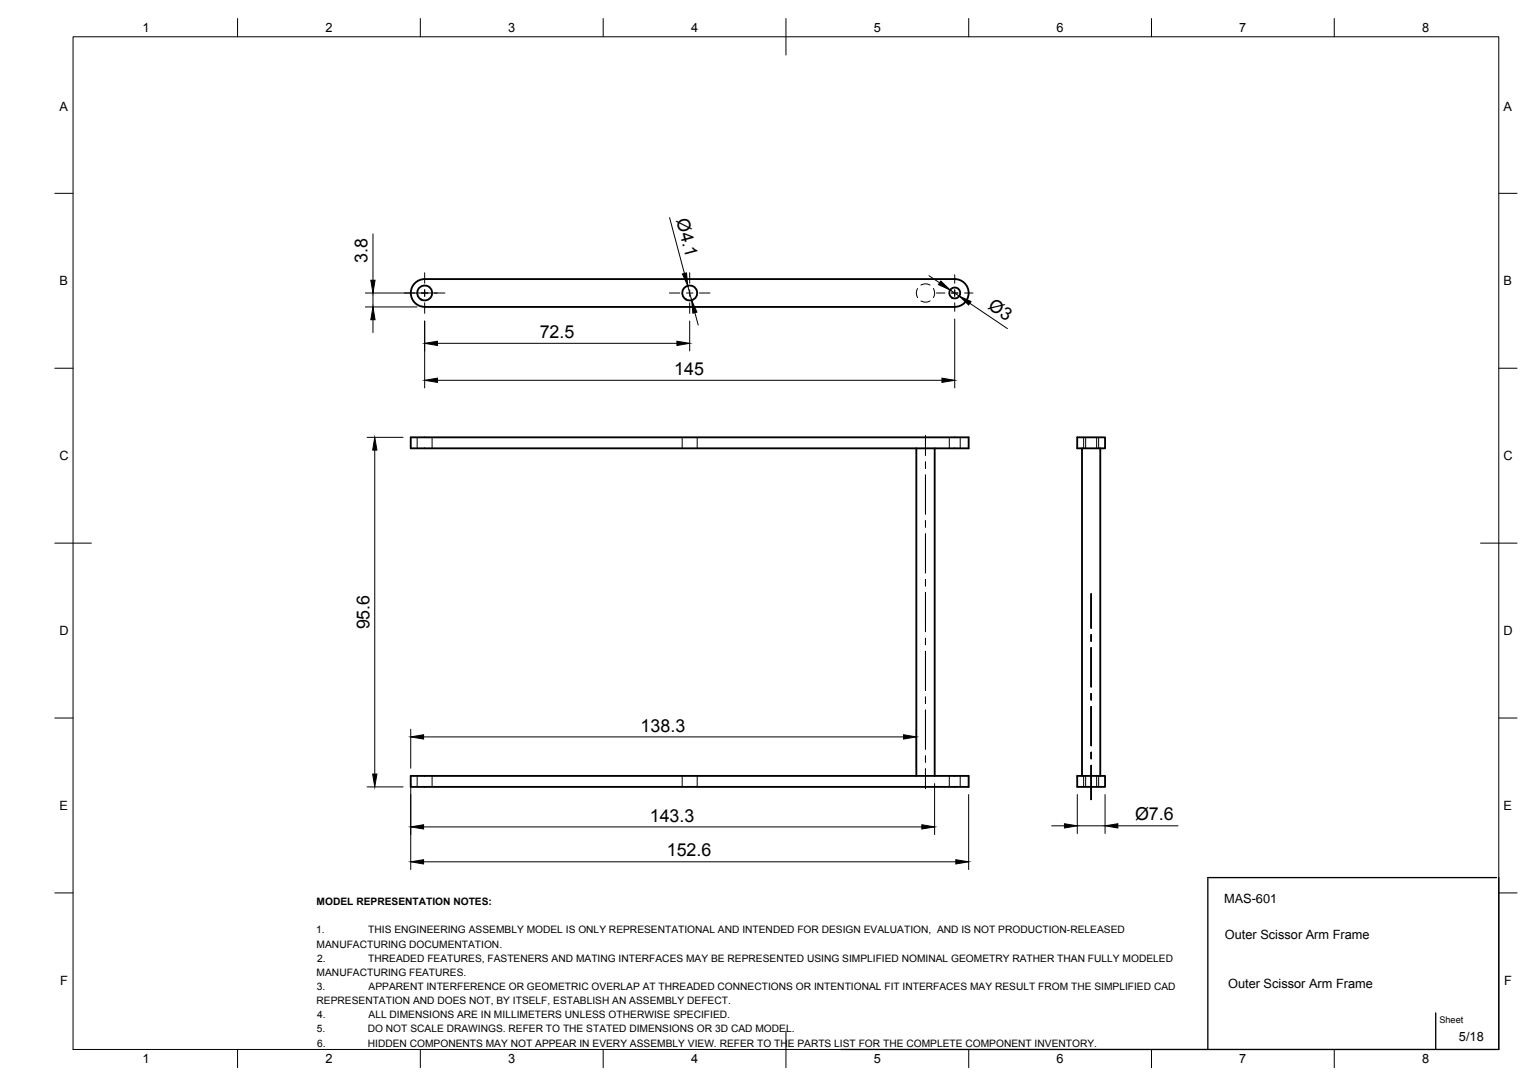
ISO-10303-21;
HEADER;
FILE_DESCRIPTION((''),'2;1');
FILE_NAME('Outer Scissor Arm Frame.step','2026-10-06T07:37:42+05:00',(''),(''),'','','');
FILE_SCHEMA (('AUTOMOTIVE_DESIGN { 1 0 10303 214 3 1 1 }'));
ENDSEC;
DATA;
#10=MECHANICAL_DESIGN_GEOMETRIC_PRESENTATION_REPRESENTATION('',(#375),#18757);
#341=SHAPE_REPRESENTATION_RELATIONSHIP('SRR','None',#18859,#358) ;
#358=ADVANCED_BREP_SHAPE_REPRESENTATION('',(#392),#18742) ;
#375=STYLED_ITEM('',(#18953),#392) ;
#392=MANIFOLD_SOLID_BREP('Outer Scissor Arm Frame',#9544) ;
#538=CYLINDRICAL_SURFACE('',#9984,2.5) ;
#539=CYLINDRICAL_SURFACE('',#9987,1.5) ;
#540=CYLINDRICAL_SURFACE('',#9990,2.05) ;
#541=CYLINDRICAL_SURFACE('',#9993,2.05) ;
#542=CYLINDRICAL_SURFACE('',#9997,3.8) ;
#543=CYLINDRICAL_SURFACE('',#10001,3.8) ;
#544=CYLINDRICAL_SURFACE('',#10006,1.5) ;
#545=CYLINDRICAL_SURFACE('',#10009,2.05) ;
#546=CYLINDRICAL_SURFACE('',#10012,2.05) ;
#547=CYLINDRICAL_SURFACE('',#10016,3.8) ;
#548=CYLINDRICAL_SURFACE('',#10020,3.8) ;
#682=FACE_BOUND('',#1785,.T.) ;
#683=FACE_BOUND('',#1786,.T.) ;
#684=FACE_BOUND('',#1787,.T.) ;
#685=FACE_BOUND('',#1788,.T.) ;
#686=FACE_BOUND('',#1790,.T.) ;
#687=FACE_BOUND('',#1791,.T.) ;
#688=FACE_BOUND('',#1792,.T.) ;
#689=FACE_BOUND('',#1801,.T.) ;
#690=FACE_BOUND('',#1802,.T.) ;
#691=FACE_BOUND('',#1803,.T.) ;
#692=FACE_BOUND('',#1805,.T.) ;
#693=FACE_BOUND('',#1806,.T.) ;
#694=FACE_BOUND('',#1807,.T.) ;
#695=FACE_BOUND('',#1808,.T.) ;
#840=PLANE('',#9996) ;
#841=PLANE('',#10000) ;
#842=PLANE('',#10004) ;
#843=PLANE('',#10005) ;
#844=PLANE('',#10015) ;
#845=PLANE('',#10019) ;
#846=PLANE('',#10023) ;
#847=PLANE('',#10024) ;
#1226=FACE_OUTER_BOUND('',#1776,.T.) ;
#1227=FACE_OUTER_BOUND('',#1777,.T.) ;
#1228=FACE_OUTER_BOUND('',#1778,.T.) ;
#1229=FACE_OUTER_BOUND('',#1779,.T.) ;
#1230=FACE_OUTER_BOUND('',#1780,.T.) ;
#1231=FACE_OUTER_BOUND('',#1781,.T.) ;
#1232=FACE_OUTER_BOUND('',#1782,.T.) ;
#1233=FACE_OUTER_BOUND('',#1783,.T.) ;
#1234=FACE_OUTER_BOUND('',#1784,.T.) ;
#1235=FACE_OUTER_BOUND('',#1789,.T.) ;
#1236=FACE_OUTER_BOUND('',#1793,.T.) ;
#1237=FACE_OUTER_BOUND('',#1794,.T.) ;
#1238=FACE_OUTER_BOUND('',#1795,.T.) ;
#1239=FACE_OUTER_BOUND('',#1796,.T.) ;
#1240=FACE_OUTER_BOUND('',#1797,.T.) ;
#1241=FACE_OUTER_BOUND('',#1798,.T.) ;
#1242=FACE_OUTER_BOUND('',#1799,.T.) ;
#1243=FACE_OUTER_BOUND('',#1800,.T.) ;
#1244=FACE_OUTER_BOUND('',#1804,.T.) ;
#1776=EDGE_LOOP('',(#7071,#7072,#7073,#7074)) ;
#1777=EDGE_LOOP('',(#7075,#7076,#7077,#7078)) ;
#1778=EDGE_LOOP('',(#7079,#7080,#7081,#7082)) ;
#1779=EDGE_LOOP('',(#7083,#7084,#7085,#7086)) ;
#1780=EDGE_LOOP('',(#7087,#7088,#7089,#7090)) ;
#1781=EDGE_LOOP('',(#7091,#7092,#7093,#7094)) ;
#1782=EDGE_LOOP('',(#7095,#7096,#7097,#7098)) ;
#1783=EDGE_LOOP('',(#7099,#7100,#7101,#7102)) ;
#1784=EDGE_LOOP('',(#7103,#7104,#7105,#7106)) ;
#1785=EDGE_LOOP('',(#7107)) ;
#1786=EDGE_LOOP('',(#7108)) ;
#1787=EDGE_LOOP('',(#7109)) ;
#1788=EDGE_LOOP('',(#7110)) ;
#1789=EDGE_LOOP('',(#7111,#7112,#7113,#7114)) ;
#1790=EDGE_LOOP('',(#7115)) ;
#1791=EDGE_LOOP('',(#7116)) ;
#1792=EDGE_LOOP('',(#7117)) ;
#1793=EDGE_LOOP('',(#7118,#7119,#7120,#7121)) ;
#1794=EDGE_LOOP('',(#7122,#7123,#7124,#7125)) ;
#1795=EDGE_LOOP('',(#7126,#7127,#7128,#7129)) ;
#1796=EDGE_LOOP('',(#7130,#7131,#7132,#7133)) ;
#1797=EDGE_LOOP('',(#7134,#7135,#7136,#7137)) ;
#1798=EDGE_LOOP('',(#7138,#7139,#7140,#7141)) ;
#1799=EDGE_LOOP('',(#7142,#7143,#7144,#7145)) ;
#1800=EDGE_LOOP('',(#7146,#7147,#7148,#7149)) ;
#1801=EDGE_LOOP('',(#7150)) ;
#1802=EDGE_LOOP('',(#7151)) ;
#1803=EDGE_LOOP('',(#7152)) ;
#1804=EDGE_LOOP('',(#7153,#7154,#7155,#7156)) ;
#1805=EDGE_LOOP('',(#7157)) ;
#1806=EDGE_LOOP('',(#7158)) ;
#1807=EDGE_LOOP('',(#7159)) ;
#1808=EDGE_LOOP('',(#7160)) ;
#2491=LINE('',#14387,#3262) ;
#2492=LINE('',#14393,#3263) ;
#2493=LINE('',#14399,#3264) ;
#2494=LINE('',#14405,#3265) ;
#2495=LINE('',#14410,#3266) ;
#2496=LINE('',#14412,#3267) ;
#2497=LINE('',#14414,#3268) ;
#2498=LINE('',#14415,#3269) ;
#2499=LINE('',#14421,#3270) ;
#2500=LINE('',#14424,#3271) ;
#2501=LINE('',#14426,#3272) ;
#2502=LINE('',#14427,#3273) ;
#2503=LINE('',#14437,#3274) ;
#2504=LINE('',#14443,#3275) ;
#2505=LINE('',#14449,#3276) ;
#2506=LINE('',#14454,#3277) ;
#2507=LINE('',#14456,#3278) ;
#2508=LINE('',#14458,#3279) ;
#2509=LINE('',#14459,#3280) ;
#2510=LINE('',#14465,#3281) ;
#2511=LINE('',#14468,#3282) ;
#2512=LINE('',#14470,#3283) ;
#2513=LINE('',#14471,#3284) ;
#3262=VECTOR('',#11451,2.5) ;
#3263=VECTOR('',#11458,1.5) ;
#3264=VECTOR('',#11465,2.05) ;
#3265=VECTOR('',#11472,2.05) ;
#3266=VECTOR('',#11477,10.) ;
#3267=VECTOR('',#11478,10.) ;
#3268=VECTOR('',#11479,10.) ;
#3269=VECTOR('',#11480,10.) ;
#3270=VECTOR('',#11487,10.) ;
#3271=VECTOR('',#11490,10.) ;
#3272=VECTOR('',#11491,10.) ;
#3273=VECTOR('',#11492,10.) ;
#3274=VECTOR('',#11507,1.5) ;
#3275=VECTOR('',#11514,2.05) ;
#3276=VECTOR('',#11521,2.05) ;
#3277=VECTOR('',#11526,10.) ;
#3278=VECTOR('',#11527,10.) ;
#3279=VECTOR('',#11528,10.) ;
#3280=VECTOR('',#11529,10.) ;
#3281=VECTOR('',#11536,10.) ;
#3282=VECTOR('',#11539,10.) ;
#3283=VECTOR('',#11540,10.) ;
#3284=VECTOR('',#11541,10.) ;
#3869=CIRCLE('',#9985,2.5) ;
#3870=CIRCLE('',#9986,2.5) ;
#3871=CIRCLE('',#9988,1.5) ;
#3872=CIRCLE('',#9989,1.5) ;
#3873=CIRCLE('',#9991,2.05) ;
#3874=CIRCLE('',#9992,2.05) ;
#3875=CIRCLE('',#9994,2.05) ;
#3876=CIRCLE('',#9995,2.05) ;
#3877=CIRCLE('',#9998,3.8) ;
#3878=CIRCLE('',#9999,3.8) ;
#3879=CIRCLE('',#10002,3.8) ;
#3880=CIRCLE('',#10003,3.8) ;
#3881=CIRCLE('',#10007,1.5) ;
#3882=CIRCLE('',#10008,1.5) ;
#3883=CIRCLE('',#10010,2.05) ;
#3884=CIRCLE('',#10011,2.05) ;
#3885=CIRCLE('',#10013,2.05) ;
#3886=CIRCLE('',#10014,2.05) ;
#3887=CIRCLE('',#10017,3.8) ;
#3888=CIRCLE('',#10018,3.8) ;
#3889=CIRCLE('',#10021,3.8) ;
#3890=CIRCLE('',#10022,3.8) ;
#4388=VERTEX_POINT('',#14384) ;
#4389=VERTEX_POINT('',#14386) ;
#4390=VERTEX_POINT('',#14390) ;
#4391=VERTEX_POINT('',#14392) ;
#4392=VERTEX_POINT('',#14396) ;
#4393=VERTEX_POINT('',#14398) ;
#4394=VERTEX_POINT('',#14402) ;
#4395=VERTEX_POINT('',#14404) ;
#4396=VERTEX_POINT('',#14408) ;
#4397=VERTEX_POINT('',#14409) ;
#4398=VERTEX_POINT('',#14411) ;
#4399=VERTEX_POINT('',#14413) ;
#4400=VERTEX_POINT('',#14417) ;
#4401=VERTEX_POINT('',#14419) ;
#4402=VERTEX_POINT('',#14423) ;
#4403=VERTEX_POINT('',#14425) ;
#4404=VERTEX_POINT('',#14434) ;
#4405=VERTEX_POINT('',#14436) ;
#4406=VERTEX_POINT('',#14440) ;
#4407=VERTEX_POINT('',#14442) ;
#4408=VERTEX_POINT('',#14446) ;
#4409=VERTEX_POINT('',#14448) ;
#4410=VERTEX_POINT('',#14452) ;
#4411=VERTEX_POINT('',#14453) ;
#4412=VERTEX_POINT('',#14455) ;
#4413=VERTEX_POINT('',#14457) ;
#4414=VERTEX_POINT('',#14461) ;
#4415=VERTEX_POINT('',#14463) ;
#4416=VERTEX_POINT('',#14467) ;
#4417=VERTEX_POINT('',#14469) ;
#5382=EDGE_CURVE('',#4388,#4388,#3869,.T.) ;
#5383=EDGE_CURVE('',#4388,#4389,#2491,.T.) ;
#5384=EDGE_CURVE('',#4389,#4389,#3870,.T.) ;
#5385=EDGE_CURVE('',#4390,#4390,#3871,.T.) ;
#5386=EDGE_CURVE('',#4390,#4391,#2492,.T.) ;
#5387=EDGE_CURVE('',#4391,#4391,#3872,.T.) ;
#5388=EDGE_CURVE('',#4392,#4392,#3873,.T.) ;
#5389=EDGE_CURVE('',#4392,#4393,#2493,.T.) ;
#5390=EDGE_CURVE('',#4393,#4393,#3874,.T.) ;
#5391=EDGE_CURVE('',#4394,#4394,#3875,.T.) ;
#5392=EDGE_CURVE('',#4394,#4395,#2494,.T.) ;
#5393=EDGE_CURVE('',#4395,#4395,#3876,.T.) ;
#5394=EDGE_CURVE('',#4396,#4397,#2495,.T.) ;
#5395=EDGE_CURVE('',#4397,#4398,#2496,.T.) ;
#5396=EDGE_CURVE('',#4399,#4398,#2497,.T.) ;
#5397=EDGE_CURVE('',#4396,#4399,#2498,.T.) ;
#5398=EDGE_CURVE('',#4400,#4396,#3877,.T.) ;
#5399=EDGE_CURVE('',#4401,#4399,#3878,.T.) ;
#5400=EDGE_CURVE('',#4400,#4401,#2499,.T.) ;
#5401=EDGE_CURVE('',#4402,#4400,#2500,.T.) ;
#5402=EDGE_CURVE('',#4403,#4401,#2501,.T.) ;
#5403=EDGE_CURVE('',#4402,#4403,#2502,.T.) ;
#5404=EDGE_CURVE('',#4397,#4402,#3879,.T.) ;
#5405=EDGE_CURVE('',#4398,#4403,#3880,.T.) ;
#5406=EDGE_CURVE('',#4404,#4404,#3881,.T.) ;
#5407=EDGE_CURVE('',#4404,#4405,#2503,.T.) ;
#5408=EDGE_CURVE('',#4405,#4405,#3882,.T.) ;
#5409=EDGE_CURVE('',#4406,#4406,#3883,.T.) ;
#5410=EDGE_CURVE('',#4406,#4407,#2504,.T.) ;
#5411=EDGE_CURVE('',#4407,#4407,#3884,.T.) ;
#5412=EDGE_CURVE('',#4408,#4408,#3885,.T.) ;
#5413=EDGE_CURVE('',#4408,#4409,#2505,.T.) ;
#5414=EDGE_CURVE('',#4409,#4409,#3886,.T.) ;
#5415=EDGE_CURVE('',#4410,#4411,#2506,.T.) ;
#5416=EDGE_CURVE('',#4411,#4412,#2507,.T.) ;
#5417=EDGE_CURVE('',#4413,#4412,#2508,.T.) ;
#5418=EDGE_CURVE('',#4410,#4413,#2509,.T.) ;
#5419=EDGE_CURVE('',#4414,#4410,#3887,.T.) ;
#5420=EDGE_CURVE('',#4415,#4413,#3888,.T.) ;
#5421=EDGE_CURVE('',#4414,#4415,#2510,.T.) ;
#5422=EDGE_CURVE('',#4416,#4414,#2511,.T.) ;
#5423=EDGE_CURVE('',#4417,#4415,#2512,.T.) ;
#5424=EDGE_CURVE('',#4416,#4417,#2513,.T.) ;
#5425=EDGE_CURVE('',#4411,#4416,#3889,.T.) ;
#5426=EDGE_CURVE('',#4412,#4417,#3890,.T.) ;
#7071=ORIENTED_EDGE('',*,*,#5382,.F.) ;
#7072=ORIENTED_EDGE('',*,*,#5383,.T.) ;
#7073=ORIENTED_EDGE('',*,*,#5384,.F.) ;
#7074=ORIENTED_EDGE('',*,*,#5383,.F.) ;
#7075=ORIENTED_EDGE('',*,*,#5385,.F.) ;
#7076=ORIENTED_EDGE('',*,*,#5386,.T.) ;
#7077=ORIENTED_EDGE('',*,*,#5387,.T.) ;
#7078=ORIENTED_EDGE('',*,*,#5386,.F.) ;
#7079=ORIENTED_EDGE('',*,*,#5388,.F.) ;
#7080=ORIENTED_EDGE('',*,*,#5389,.T.) ;
#7081=ORIENTED_EDGE('',*,*,#5390,.T.) ;
#7082=ORIENTED_EDGE('',*,*,#5389,.F.) ;
#7083=ORIENTED_EDGE('',*,*,#5391,.F.) ;
#7084=ORIENTED_EDGE('',*,*,#5392,.T.) ;
#7085=ORIENTED_EDGE('',*,*,#5393,.T.) ;
#7086=ORIENTED_EDGE('',*,*,#5392,.F.) ;
#7087=ORIENTED_EDGE('',*,*,#5394,.T.) ;
#7088=ORIENTED_EDGE('',*,*,#5395,.T.) ;
#7089=ORIENTED_EDGE('',*,*,#5396,.F.) ;
#7090=ORIENTED_EDGE('',*,*,#5397,.F.) ;
#7091=ORIENTED_EDGE('',*,*,#5398,.T.) ;
#7092=ORIENTED_EDGE('',*,*,#5397,.T.) ;
#7093=ORIENTED_EDGE('',*,*,#5399,.F.) ;
#7094=ORIENTED_EDGE('',*,*,#5400,.F.) ;
#7095=ORIENTED_EDGE('',*,*,#5401,.T.) ;
#7096=ORIENTED_EDGE('',*,*,#5400,.T.) ;
#7097=ORIENTED_EDGE('',*,*,#5402,.F.) ;
#7098=ORIENTED_EDGE('',*,*,#5403,.F.) ;
#7099=ORIENTED_EDGE('',*,*,#5404,.T.) ;
#7100=ORIENTED_EDGE('',*,*,#5403,.T.) ;
#7101=ORIENTED_EDGE('',*,*,#5405,.F.) ;
#7102=ORIENTED_EDGE('',*,*,#5395,.F.) ;
#7103=ORIENTED_EDGE('',*,*,#5405,.T.) ;
#7104=ORIENTED_EDGE('',*,*,#5402,.T.) ;
#7105=ORIENTED_EDGE('',*,*,#5399,.T.) ;
#7106=ORIENTED_EDGE('',*,*,#5396,.T.) ;
#7107=ORIENTED_EDGE('',*,*,#5384,.T.) ;
#7108=ORIENTED_EDGE('',*,*,#5391,.T.) ;
#7109=ORIENTED_EDGE('',*,*,#5388,.T.) ;
#7110=ORIENTED_EDGE('',*,*,#5385,.T.) ;
#7111=ORIENTED_EDGE('',*,*,#5404,.F.) ;
#7112=ORIENTED_EDGE('',*,*,#5394,.F.) ;
#7113=ORIENTED_EDGE('',*,*,#5398,.F.) ;
#7114=ORIENTED_EDGE('',*,*,#5401,.F.) ;
#7115=ORIENTED_EDGE('',*,*,#5393,.F.) ;
#7116=ORIENTED_EDGE('',*,*,#5390,.F.) ;
#7117=ORIENTED_EDGE('',*,*,#5387,.F.) ;
#7118=ORIENTED_EDGE('',*,*,#5406,.F.) ;
#7119=ORIENTED_EDGE('',*,*,#5407,.T.) ;
#7120=ORIENTED_EDGE('',*,*,#5408,.T.) ;
#7121=ORIENTED_EDGE('',*,*,#5407,.F.) ;
#7122=ORIENTED_EDGE('',*,*,#5409,.F.) ;
#7123=ORIENTED_EDGE('',*,*,#5410,.T.) ;
#7124=ORIENTED_EDGE('',*,*,#5411,.T.) ;
#7125=ORIENTED_EDGE('',*,*,#5410,.F.) ;
#7126=ORIENTED_EDGE('',*,*,#5412,.F.) ;
#7127=ORIENTED_EDGE('',*,*,#5413,.T.) ;
#7128=ORIENTED_EDGE('',*,*,#5414,.T.) ;
#7129=ORIENTED_EDGE('',*,*,#5413,.F.) ;
#7130=ORIENTED_EDGE('',*,*,#5415,.T.) ;
#7131=ORIENTED_EDGE('',*,*,#5416,.T.) ;
#7132=ORIENTED_EDGE('',*,*,#5417,.F.) ;
#7133=ORIENTED_EDGE('',*,*,#5418,.F.) ;
#7134=ORIENTED_EDGE('',*,*,#5419,.T.) ;
#7135=ORIENTED_EDGE('',*,*,#5418,.T.) ;
#7136=ORIENTED_EDGE('',*,*,#5420,.F.) ;
#7137=ORIENTED_EDGE('',*,*,#5421,.F.) ;
#7138=ORIENTED_EDGE('',*,*,#5422,.T.) ;
#7139=ORIENTED_EDGE('',*,*,#5421,.T.) ;
#7140=ORIENTED_EDGE('',*,*,#5423,.F.) ;
#7141=ORIENTED_EDGE('',*,*,#5424,.F.) ;
#7142=ORIENTED_EDGE('',*,*,#5425,.T.) ;
#7143=ORIENTED_EDGE('',*,*,#5424,.T.) ;
#7144=ORIENTED_EDGE('',*,*,#5426,.F.) ;
#7145=ORIENTED_EDGE('',*,*,#5416,.F.) ;
#7146=ORIENTED_EDGE('',*,*,#5426,.T.) ;
#7147=ORIENTED_EDGE('',*,*,#5423,.T.) ;
#7148=ORIENTED_EDGE('',*,*,#5420,.T.) ;
#7149=ORIENTED_EDGE('',*,*,#5417,.T.) ;
#7150=ORIENTED_EDGE('',*,*,#5412,.T.) ;
#7151=ORIENTED_EDGE('',*,*,#5409,.T.) ;
#7152=ORIENTED_EDGE('',*,*,#5406,.T.) ;
#7153=ORIENTED_EDGE('',*,*,#5425,.F.) ;
#7154=ORIENTED_EDGE('',*,*,#5415,.F.) ;
#7155=ORIENTED_EDGE('',*,*,#5419,.F.) ;
#7156=ORIENTED_EDGE('',*,*,#5422,.F.) ;
#7157=ORIENTED_EDGE('',*,*,#5382,.T.) ;
#7158=ORIENTED_EDGE('',*,*,#5414,.F.) ;
#7159=ORIENTED_EDGE('',*,*,#5411,.F.) ;
#7160=ORIENTED_EDGE('',*,*,#5408,.F.) ;
#9162=ADVANCED_FACE('',(#1226),#538,.T.) ;
#9163=ADVANCED_FACE('',(#1227),#539,.F.) ;
#9164=ADVANCED_FACE('',(#1228),#540,.F.) ;
#9165=ADVANCED_FACE('',(#1229),#541,.F.) ;
#9166=ADVANCED_FACE('',(#1230),#840,.T.) ;
#9167=ADVANCED_FACE('',(#1231),#542,.T.) ;
#9168=ADVANCED_FACE('',(#1232),#841,.T.) ;
#9169=ADVANCED_FACE('',(#1233),#543,.T.) ;
#9170=ADVANCED_FACE('',(#1234,#682,#683,#684,#685),#842,.T.) ;
#9171=ADVANCED_FACE('',(#1235,#686,#687,#688),#843,.F.) ;
#9172=ADVANCED_FACE('',(#1236),#544,.F.) ;
#9173=ADVANCED_FACE('',(#1237),#545,.F.) ;
#9174=ADVANCED_FACE('',(#1238),#546,.F.) ;
#9175=ADVANCED_FACE('',(#1239),#844,.T.) ;
#9176=ADVANCED_FACE('',(#1240),#547,.T.) ;
#9177=ADVANCED_FACE('',(#1241),#845,.T.) ;
#9178=ADVANCED_FACE('',(#1242),#548,.T.) ;
#9179=ADVANCED_FACE('',(#1243,#689,#690,#691),#846,.T.) ;
#9180=ADVANCED_FACE('',(#1244,#692,#693,#694,#695),#847,.F.) ;
#9544=CLOSED_SHELL('',(#9162,#9163,#9164,#9165,#9166,#9167,#9168,#9169,
#9170,#9171,#9172,#9173,#9174,#9175,#9176,#9177,#9178,#9179,#9180)) ;
#9983=AXIS2_PLACEMENT_3D('',#14382,#11445,#11446) ;
#9984=AXIS2_PLACEMENT_3D('',#14383,#11447,#11448) ;
#9985=AXIS2_PLACEMENT_3D('',#14385,#11449,#11450) ;
#9986=AXIS2_PLACEMENT_3D('',#14388,#11452,#11453) ;
#9987=AXIS2_PLACEMENT_3D('',#14389,#11454,#11455) ;
#9988=AXIS2_PLACEMENT_3D('',#14391,#11456,#11457) ;
#9989=AXIS2_PLACEMENT_3D('',#14394,#11459,#11460) ;
#9990=AXIS2_PLACEMENT_3D('',#14395,#11461,#11462) ;
#9991=AXIS2_PLACEMENT_3D('',#14397,#11463,#11464) ;
#9992=AXIS2_PLACEMENT_3D('',#14400,#11466,#11467) ;
#9993=AXIS2_PLACEMENT_3D('',#14401,#11468,#11469) ;
#9994=AXIS2_PLACEMENT_3D('',#14403,#11470,#11471) ;
#9995=AXIS2_PLACEMENT_3D('',#14406,#11473,#11474) ;
#9996=AXIS2_PLACEMENT_3D('',#14407,#11475,#11476) ;
#9997=AXIS2_PLACEMENT_3D('',#14416,#11481,#11482) ;
#9998=AXIS2_PLACEMENT_3D('',#14418,#11483,#11484) ;
#9999=AXIS2_PLACEMENT_3D('',#14420,#11485,#11486) ;
#10000=AXIS2_PLACEMENT_3D('',#14422,#11488,#11489) ;
#10001=AXIS2_PLACEMENT_3D('',#14428,#11493,#11494) ;
#10002=AXIS2_PLACEMENT_3D('',#14429,#11495,#11496) ;
#10003=AXIS2_PLACEMENT_3D('',#14430,#11497,#11498) ;
#10004=AXIS2_PLACEMENT_3D('',#14431,#11499,#11500) ;
#10005=AXIS2_PLACEMENT_3D('',#14432,#11501,#11502) ;
#10006=AXIS2_PLACEMENT_3D('',#14433,#11503,#11504) ;
#10007=AXIS2_PLACEMENT_3D('',#14435,#11505,#11506) ;
#10008=AXIS2_PLACEMENT_3D('',#14438,#11508,#11509) ;
#10009=AXIS2_PLACEMENT_3D('',#14439,#11510,#11511) ;
#10010=AXIS2_PLACEMENT_3D('',#14441,#11512,#11513) ;
#10011=AXIS2_PLACEMENT_3D('',#14444,#11515,#11516) ;
#10012=AXIS2_PLACEMENT_3D('',#14445,#11517,#11518) ;
#10013=AXIS2_PLACEMENT_3D('',#14447,#11519,#11520) ;
#10014=AXIS2_PLACEMENT_3D('',#14450,#11522,#11523) ;
#10015=AXIS2_PLACEMENT_3D('',#14451,#11524,#11525) ;
#10016=AXIS2_PLACEMENT_3D('',#14460,#11530,#11531) ;
#10017=AXIS2_PLACEMENT_3D('',#14462,#11532,#11533) ;
#10018=AXIS2_PLACEMENT_3D('',#14464,#11534,#11535) ;
#10019=AXIS2_PLACEMENT_3D('',#14466,#11537,#11538) ;
#10020=AXIS2_PLACEMENT_3D('',#14472,#11542,#11543) ;
#10021=AXIS2_PLACEMENT_3D('',#14473,#11544,#11545) ;
#10022=AXIS2_PLACEMENT_3D('',#14474,#11546,#11547) ;
#10023=AXIS2_PLACEMENT_3D('',#14475,#11548,#11549) ;
#10024=AXIS2_PLACEMENT_3D('',#14476,#11550,#11551) ;
#11445=DIRECTION('axis',(0.,0.,1.)) ;
#11446=DIRECTION('refdir',(1.,0.,0.)) ;
#11447=DIRECTION('center_axis',(0.,1.,0.)) ;
#11448=DIRECTION('ref_axis',(1.,0.,0.)) ;
#11449=DIRECTION('center_axis',(0.,1.,0.)) ;
#11450=DIRECTION('ref_axis',(1.,0.,0.)) ;
#11451=DIRECTION('',(0.,-1.,0.)) ;
#11452=DIRECTION('center_axis',(0.,-1.,0.)) ;
#11453=DIRECTION('ref_axis',(1.,0.,0.)) ;
#11454=DIRECTION('center_axis',(0.,1.,0.)) ;
#11455=DIRECTION('ref_axis',(1.,0.,0.)) ;
#11456=DIRECTION('center_axis',(0.,-1.,0.)) ;
#11457=DIRECTION('ref_axis',(1.,0.,0.)) ;
#11458=DIRECTION('',(0.,-1.,0.)) ;
#11459=DIRECTION('center_axis',(0.,-1.,0.)) ;
#11460=DIRECTION('ref_axis',(1.,0.,0.)) ;
#11461=DIRECTION('center_axis',(0.,1.,0.)) ;
#11462=DIRECTION('ref_axis',(1.,0.,0.)) ;
#11463=DIRECTION('center_axis',(0.,-1.,0.)) ;
#11464=DIRECTION('ref_axis',(1.,0.,0.)) ;
#11465=DIRECTION('',(0.,-1.,0.)) ;
#11466=DIRECTION('center_axis',(0.,-1.,0.)) ;
#11467=DIRECTION('ref_axis',(1.,0.,0.)) ;
#11468=DIRECTION('center_axis',(0.,1.,0.)) ;
#11469=DIRECTION('ref_axis',(1.,0.,0.)) ;
#11470=DIRECTION('center_axis',(0.,-1.,0.)) ;
#11471=DIRECTION('ref_axis',(1.,0.,0.)) ;
#11472=DIRECTION('',(0.,-1.,0.)) ;
#11473=DIRECTION('center_axis',(0.,-1.,0.)) ;
#11474=DIRECTION('ref_axis',(1.,0.,0.)) ;
#11475=DIRECTION('center_axis',(0.0648275862068965,0.,0.997896479634329)) ;
#11476=DIRECTION('ref_axis',(0.997896479634329,0.,-0.0648275862068965)) ;
#11477=DIRECTION('',(0.997896479634329,0.,-0.0648275862068965)) ;
#11478=DIRECTION('',(0.,1.,0.)) ;
#11479=DIRECTION('',(0.997896479634329,0.,-0.0648275862068965)) ;
#11480=DIRECTION('',(0.,1.,0.)) ;
#11481=DIRECTION('center_axis',(0.,1.,0.)) ;
#11482=DIRECTION('ref_axis',(-0.0648275862068983,0.,-0.997896479634329)) ;
#11483=DIRECTION('center_axis',(0.,1.,0.)) ;
#11484=DIRECTION('ref_axis',(-0.0648275862068983,0.,-0.997896479634329)) ;
#11485=DIRECTION('center_axis',(0.,1.,0.)) ;
#11486=DIRECTION('ref_axis',(-0.0648275862068983,0.,-0.997896479634329)) ;
#11487=DIRECTION('',(0.,1.,0.)) ;
#11488=DIRECTION('center_axis',(-0.0648275862068965,0.,-0.997896479634329)) ;
#11489=DIRECTION('ref_axis',(-0.997896479634329,0.,0.0648275862068965)) ;
#11490=DIRECTION('',(-0.997896479634329,0.,0.0648275862068965)) ;
#11491=DIRECTION('',(-0.997896479634329,0.,0.0648275862068965)) ;
#11492=DIRECTION('',(0.,1.,0.)) ;
#11493=DIRECTION('center_axis',(0.,1.,0.)) ;
#11494=DIRECTION('ref_axis',(0.064827586206896,0.,0.997896479634329)) ;
#11495=DIRECTION('center_axis',(0.,1.,0.)) ;
#11496=DIRECTION('ref_axis',(0.064827586206896,0.,0.997896479634329)) ;
#11497=DIRECTION('center_axis',(0.,1.,0.)) ;
#11498=DIRECTION('ref_axis',(0.064827586206896,0.,0.997896479634329)) ;
#11499=DIRECTION('center_axis',(0.,1.,0.)) ;
#11500=DIRECTION('ref_axis',(1.,0.,0.)) ;
#11501=DIRECTION('center_axis',(0.,1.,0.)) ;
#11502=DIRECTION('ref_axis',(1.,0.,0.)) ;
#11503=DIRECTION('center_axis',(0.,1.,0.)) ;
#11504=DIRECTION('ref_axis',(1.,0.,0.)) ;
#11505=DIRECTION('center_axis',(0.,-1.,0.)) ;
#11506=DIRECTION('ref_axis',(1.,0.,0.)) ;
#11507=DIRECTION('',(0.,-1.,0.)) ;
#11508=DIRECTION('center_axis',(0.,-1.,0.)) ;
#11509=DIRECTION('ref_axis',(1.,0.,0.)) ;
#11510=DIRECTION('center_axis',(0.,1.,0.)) ;
#11511=DIRECTION('ref_axis',(1.,0.,0.)) ;
#11512=DIRECTION('center_axis',(0.,-1.,0.)) ;
#11513=DIRECTION('ref_axis',(1.,0.,0.)) ;
#11514=DIRECTION('',(0.,-1.,0.)) ;
#11515=DIRECTION('center_axis',(0.,-1.,0.)) ;
#11516=DIRECTION('ref_axis',(1.,0.,0.)) ;
#11517=DIRECTION('center_axis',(0.,1.,0.)) ;
#11518=DIRECTION('ref_axis',(1.,0.,0.)) ;
#11519=DIRECTION('center_axis',(0.,-1.,0.)) ;
#11520=DIRECTION('ref_axis',(1.,0.,0.)) ;
#11521=DIRECTION('',(0.,-1.,0.)) ;
#11522=DIRECTION('center_axis',(0.,-1.,0.)) ;
#11523=DIRECTION('ref_axis',(1.,0.,0.)) ;
#11524=DIRECTION('center_axis',(0.0648275862068965,0.,0.997896479634329)) ;
#11525=DIRECTION('ref_axis',(0.997896479634329,0.,-0.0648275862068965)) ;
#11526=DIRECTION('',(0.997896479634329,0.,-0.0648275862068965)) ;
#11527=DIRECTION('',(0.,1.,0.)) ;
#11528=DIRECTION('',(0.997896479634329,0.,-0.0648275862068965)) ;
#11529=DIRECTION('',(0.,1.,0.)) ;
#11530=DIRECTION('center_axis',(0.,1.,0.)) ;
#11531=DIRECTION('ref_axis',(-0.0648275862068983,0.,-0.997896479634329)) ;
#11532=DIRECTION('center_axis',(0.,1.,0.)) ;
#11533=DIRECTION('ref_axis',(-0.0648275862068983,0.,-0.997896479634329)) ;
#11534=DIRECTION('center_axis',(0.,1.,0.)) ;
#11535=DIRECTION('ref_axis',(-0.0648275862068983,0.,-0.997896479634329)) ;
#11536=DIRECTION('',(0.,1.,0.)) ;
#11537=DIRECTION('center_axis',(-0.0648275862068965,0.,-0.997896479634329)) ;
#11538=DIRECTION('ref_axis',(-0.997896479634329,0.,0.0648275862068965)) ;
#11539=DIRECTION('',(-0.997896479634329,0.,0.0648275862068965)) ;
#11540=DIRECTION('',(-0.997896479634329,0.,0.0648275862068965)) ;
#11541=DIRECTION('',(0.,1.,0.)) ;
#11542=DIRECTION('center_axis',(0.,1.,0.)) ;
#11543=DIRECTION('ref_axis',(0.064827586206896,0.,0.997896479634329)) ;
#11544=DIRECTION('center_axis',(0.,1.,0.)) ;
#11545=DIRECTION('ref_axis',(0.064827586206896,0.,0.997896479634329)) ;
#11546=DIRECTION('center_axis',(0.,1.,0.)) ;
#11547=DIRECTION('ref_axis',(0.064827586206896,0.,0.997896479634329)) ;
#11548=DIRECTION('center_axis',(0.,1.,0.)) ;
#11549=DIRECTION('ref_axis',(1.,0.,0.)) ;
#11550=DIRECTION('center_axis',(0.,1.,0.)) ;
#11551=DIRECTION('ref_axis',(1.,0.,0.)) ;
#14382=CARTESIAN_POINT('',(0.,0.,0.)) ;
#14383=CARTESIAN_POINT('Origin',(-64.7118177099031,-45.3,43.8813793103448)) ;
#14384=CARTESIAN_POINT('',(-67.2118177099031,44.8,43.8813793103448)) ;
#14385=CARTESIAN_POINT('Origin',(-64.7118177099031,44.8,43.8813793103448)) ;
#14386=CARTESIAN_POINT('',(-67.2118177099031,-44.8,43.8813793103448)) ;
#14387=CARTESIAN_POINT('',(-67.2118177099031,-45.3,43.8813793103448)) ;
#14388=CARTESIAN_POINT('Origin',(-64.7118177099031,-44.8,43.8813793103448)) ;
#14389=CARTESIAN_POINT('Origin',(-72.6949895469778,-47.8,44.4)) ;
#14390=CARTESIAN_POINT('',(-74.1949895469778,-44.8,44.4)) ;
#14391=CARTESIAN_POINT('Origin',(-72.6949895469778,-44.8,44.4)) ;
#14392=CARTESIAN_POINT('',(-74.1949895469778,-47.8,44.4)) ;
#14393=CARTESIAN_POINT('',(-74.1949895469778,-47.8,44.4)) ;
#14394=CARTESIAN_POINT('Origin',(-72.6949895469778,-47.8,44.4)) ;
#14395=CARTESIAN_POINT('Origin',(-0.347494773488876,-47.8,39.7)) ;
#14396=CARTESIAN_POINT('',(-2.39749477348887,-44.8,39.7)) ;
#14397=CARTESIAN_POINT('Origin',(-0.347494773488876,-44.8,39.7)) ;
#14398=CARTESIAN_POINT('',(-2.39749477348888,-47.8,39.7)) ;
#14399=CARTESIAN_POINT('',(-2.39749477348888,-47.8,39.7)) ;
#14400=CARTESIAN_POINT('Origin',(-0.347494773488876,-47.8,39.7)) ;
#14401=CARTESIAN_POINT('Origin',(72.,-47.8,35.)) ;
#14402=CARTESIAN_POINT('',(69.95,-44.8,35.)) ;
#14403=CARTESIAN_POINT('Origin',(72.,-44.8,35.)) ;
#14404=CARTESIAN_POINT('',(69.95,-47.8,35.)) ;
#14405=CARTESIAN_POINT('',(69.95,-47.8,35.)) ;
#14406=CARTESIAN_POINT('Origin',(72.,-47.8,35.)) ;
#14407=CARTESIAN_POINT('Origin',(-72.4486447193915,-47.8,48.1920066226104)) ;
#14408=CARTESIAN_POINT('',(-72.4486447193915,-47.8,48.1920066226104)) ;
#14409=CARTESIAN_POINT('',(72.2463448275862,-47.8,38.7920066226105)) ;
#14410=CARTESIAN_POINT('',(-72.4486447193915,-47.8,48.1920066226104)) ;
#14411=CARTESIAN_POINT('',(72.2463448275862,-44.8,38.7920066226105)) ;
#14412=CARTESIAN_POINT('',(72.2463448275862,-47.8,38.7920066226105)) ;
#14413=CARTESIAN_POINT('',(-72.4486447193915,-44.8,48.1920066226104)) ;
#14414=CARTESIAN_POINT('',(-72.4486447193915,-44.8,48.1920066226104)) ;
#14415=CARTESIAN_POINT('',(-72.4486447193915,-47.8,48.1920066226104)) ;
#14416=CARTESIAN_POINT('Origin',(-72.6949895469778,-47.8,44.4)) ;
#14417=CARTESIAN_POINT('',(-72.941334374564,-47.8,40.6079933773895)) ;
#14418=CARTESIAN_POINT('Origin',(-72.6949895469778,-47.8,44.4)) ;
#14419=CARTESIAN_POINT('',(-72.941334374564,-44.8,40.6079933773895)) ;
#14420=CARTESIAN_POINT('Origin',(-72.6949895469778,-44.8,44.4)) ;
#14421=CARTESIAN_POINT('',(-72.941334374564,-47.8,40.6079933773895)) ;
#14422=CARTESIAN_POINT('Origin',(71.7536551724138,-47.8,31.2079933773895)) ;
#14423=CARTESIAN_POINT('',(71.7536551724138,-47.8,31.2079933773895)) ;
#14424=CARTESIAN_POINT('',(71.7536551724138,-47.8,31.2079933773895)) ;
#14425=CARTESIAN_POINT('',(71.7536551724138,-44.8,31.2079933773895)) ;
#14426=CARTESIAN_POINT('',(71.7536551724138,-44.8,31.2079933773895)) ;
#14427=CARTESIAN_POINT('',(71.7536551724138,-47.8,31.2079933773895)) ;
#14428=CARTESIAN_POINT('Origin',(72.,-47.8,35.)) ;
#14429=CARTESIAN_POINT('Origin',(72.,-47.8,35.)) ;
#14430=CARTESIAN_POINT('Origin',(72.,-44.8,35.)) ;
#14431=CARTESIAN_POINT('Origin',(-0.347494773488872,-44.8,39.7)) ;
#14432=CARTESIAN_POINT('Origin',(-0.347494773488872,-47.8,39.7)) ;
#14433=CARTESIAN_POINT('Origin',(-72.6949895469778,44.8,44.4)) ;
#14434=CARTESIAN_POINT('',(-74.1949895469778,47.8,44.4)) ;
#14435=CARTESIAN_POINT('Origin',(-72.6949895469778,47.8,44.4)) ;
#14436=CARTESIAN_POINT('',(-74.1949895469778,44.8,44.4)) ;
#14437=CARTESIAN_POINT('',(-74.1949895469778,44.8,44.4)) ;
#14438=CARTESIAN_POINT('Origin',(-72.6949895469778,44.8,44.4)) ;
#14439=CARTESIAN_POINT('Origin',(-0.347494773488876,44.8,39.7)) ;
#14440=CARTESIAN_POINT('',(-2.39749477348887,47.8,39.7)) ;
#14441=CARTESIAN_POINT('Origin',(-0.347494773488876,47.8,39.7)) ;
#14442=CARTESIAN_POINT('',(-2.39749477348888,44.8,39.7)) ;
#14443=CARTESIAN_POINT('',(-2.39749477348888,44.8,39.7)) ;
#14444=CARTESIAN_POINT('Origin',(-0.347494773488876,44.8,39.7)) ;
#14445=CARTESIAN_POINT('Origin',(72.,44.8,35.)) ;
#14446=CARTESIAN_POINT('',(69.95,47.8,35.)) ;
#14447=CARTESIAN_POINT('Origin',(72.,47.8,35.)) ;
#14448=CARTESIAN_POINT('',(69.95,44.8,35.)) ;
#14449=CARTESIAN_POINT('',(69.95,44.8,35.)) ;
#14450=CARTESIAN_POINT('Origin',(72.,44.8,35.)) ;
#14451=CARTESIAN_POINT('Origin',(-72.4486447193915,44.8,48.1920066226104)) ;
#14452=CARTESIAN_POINT('',(-72.4486447193915,44.8,48.1920066226104)) ;
#14453=CARTESIAN_POINT('',(72.2463448275862,44.8,38.7920066226105)) ;
#14454=CARTESIAN_POINT('',(-72.4486447193915,44.8,48.1920066226104)) ;
#14455=CARTESIAN_POINT('',(72.2463448275862,47.8,38.7920066226105)) ;
#14456=CARTESIAN_POINT('',(72.2463448275862,44.8,38.7920066226105)) ;
#14457=CARTESIAN_POINT('',(-72.4486447193915,47.8,48.1920066226104)) ;
#14458=CARTESIAN_POINT('',(-72.4486447193915,47.8,48.1920066226104)) ;
#14459=CARTESIAN_POINT('',(-72.4486447193915,44.8,48.1920066226104)) ;
#14460=CARTESIAN_POINT('Origin',(-72.6949895469778,44.8,44.4)) ;
#14461=CARTESIAN_POINT('',(-72.941334374564,44.8,40.6079933773895)) ;
#14462=CARTESIAN_POINT('Origin',(-72.6949895469778,44.8,44.4)) ;
#14463=CARTESIAN_POINT('',(-72.941334374564,47.8,40.6079933773895)) ;
#14464=CARTESIAN_POINT('Origin',(-72.6949895469778,47.8,44.4)) ;
#14465=CARTESIAN_POINT('',(-72.941334374564,44.8,40.6079933773895)) ;
#14466=CARTESIAN_POINT('Origin',(71.7536551724138,44.8,31.2079933773895)) ;
#14467=CARTESIAN_POINT('',(71.7536551724138,44.8,31.2079933773895)) ;
#14468=CARTESIAN_POINT('',(71.7536551724138,44.8,31.2079933773895)) ;
#14469=CARTESIAN_POINT('',(71.7536551724138,47.8,31.2079933773895)) ;
#14470=CARTESIAN_POINT('',(71.7536551724138,47.8,31.2079933773895)) ;
#14471=CARTESIAN_POINT('',(71.7536551724138,44.8,31.2079933773895)) ;
#14472=CARTESIAN_POINT('Origin',(72.,44.8,35.)) ;
#14473=CARTESIAN_POINT('Origin',(72.,44.8,35.)) ;
#14474=CARTESIAN_POINT('Origin',(72.,47.8,35.)) ;
#14475=CARTESIAN_POINT('Origin',(-0.347494773488872,47.8,39.7)) ;
#14476=CARTESIAN_POINT('Origin',(-0.347494773488872,44.8,39.7)) ;
#18723=UNCERTAINTY_MEASURE_WITH_UNIT(LENGTH_MEASURE(0.01),#18758,
'DISTANCE_ACCURACY_VALUE',
'Maximum model space distance between geometric entities at asserted c
onnectivities') ;
#18738=UNCERTAINTY_MEASURE_WITH_UNIT(LENGTH_MEASURE(0.01),#18758,
'DISTANCE_ACCURACY_VALUE',
'Maximum model space distance between geometric entities at asserted c
onnectivities') ;
#18742=(
GEOMETRIC_REPRESENTATION_CONTEXT(3)
GLOBAL_UNCERTAINTY_ASSIGNED_CONTEXT((#18723))
GLOBAL_UNIT_ASSIGNED_CONTEXT((#18758,#18760,#18761))
REPRESENTATION_CONTEXT('','3D')
) ;
#18757=(
GEOMETRIC_REPRESENTATION_CONTEXT(3)
GLOBAL_UNCERTAINTY_ASSIGNED_CONTEXT((#18738))
GLOBAL_UNIT_ASSIGNED_CONTEXT((#18758,#18760,#18761))
REPRESENTATION_CONTEXT('','3D')
) ;
#18758=(
LENGTH_UNIT()
NAMED_UNIT(*)
SI_UNIT(.MILLI.,.METRE.)
) ;
#18760=(
NAMED_UNIT(*)
PLANE_ANGLE_UNIT()
SI_UNIT($,.RADIAN.)
) ;
#18761=(
NAMED_UNIT(*)
SI_UNIT($,.STERADIAN.)
SOLID_ANGLE_UNIT()
) ;
#18765=SHAPE_DEFINITION_REPRESENTATION(#18783,#18859) ;
#18783=PRODUCT_DEFINITION_SHAPE('',$,#18878) ;
#18859=SHAPE_REPRESENTATION('',(#9983),#18742) ;
#18874=PRODUCT_DEFINITION_CONTEXT('part definition',#18930,'design') ;
#18878=PRODUCT_DEFINITION('Outer Scissor Arm Frame',
'Outer Scissor Arm Frame',#18896,#18874) ;
#18896=PRODUCT_DEFINITION_FORMATION('',$,#18935) ;
#18930=APPLICATION_CONTEXT(
'Core Data for Automotive Mechanical Design Process') ;
#18931=PRODUCT_CONTEXT('part definition',#18930,'mechanical') ;
#18935=PRODUCT('Outer Scissor Arm Frame','Outer Scissor Arm Frame',$,(#18931)) ;
#18953=PRESENTATION_STYLE_ASSIGNMENT((#18971)) ;
#18971=SURFACE_STYLE_USAGE(.BOTH.,#18989) ;
#18989=SURFACE_SIDE_STYLE('',(#19007)) ;
#19007=SURFACE_STYLE_FILL_AREA(#19025) ;
#19025=FILL_AREA_STYLE(
'MAS-253 Metallic Sheet - Outer Scissor Arm Frame',(#19043)) ;
#19043=FILL_AREA_STYLE_COLOUR(
'MAS-253 Metallic Sheet - Outer Scissor Arm Frame',#19061) ;
#19061=COLOUR_RGB('MAS-253 Metallic Sheet - Outer Scissor Arm Frame', 0.40784314, 0.44705882, 0.49803922) ;
ENDSEC;
END-ISO-10303-21;
